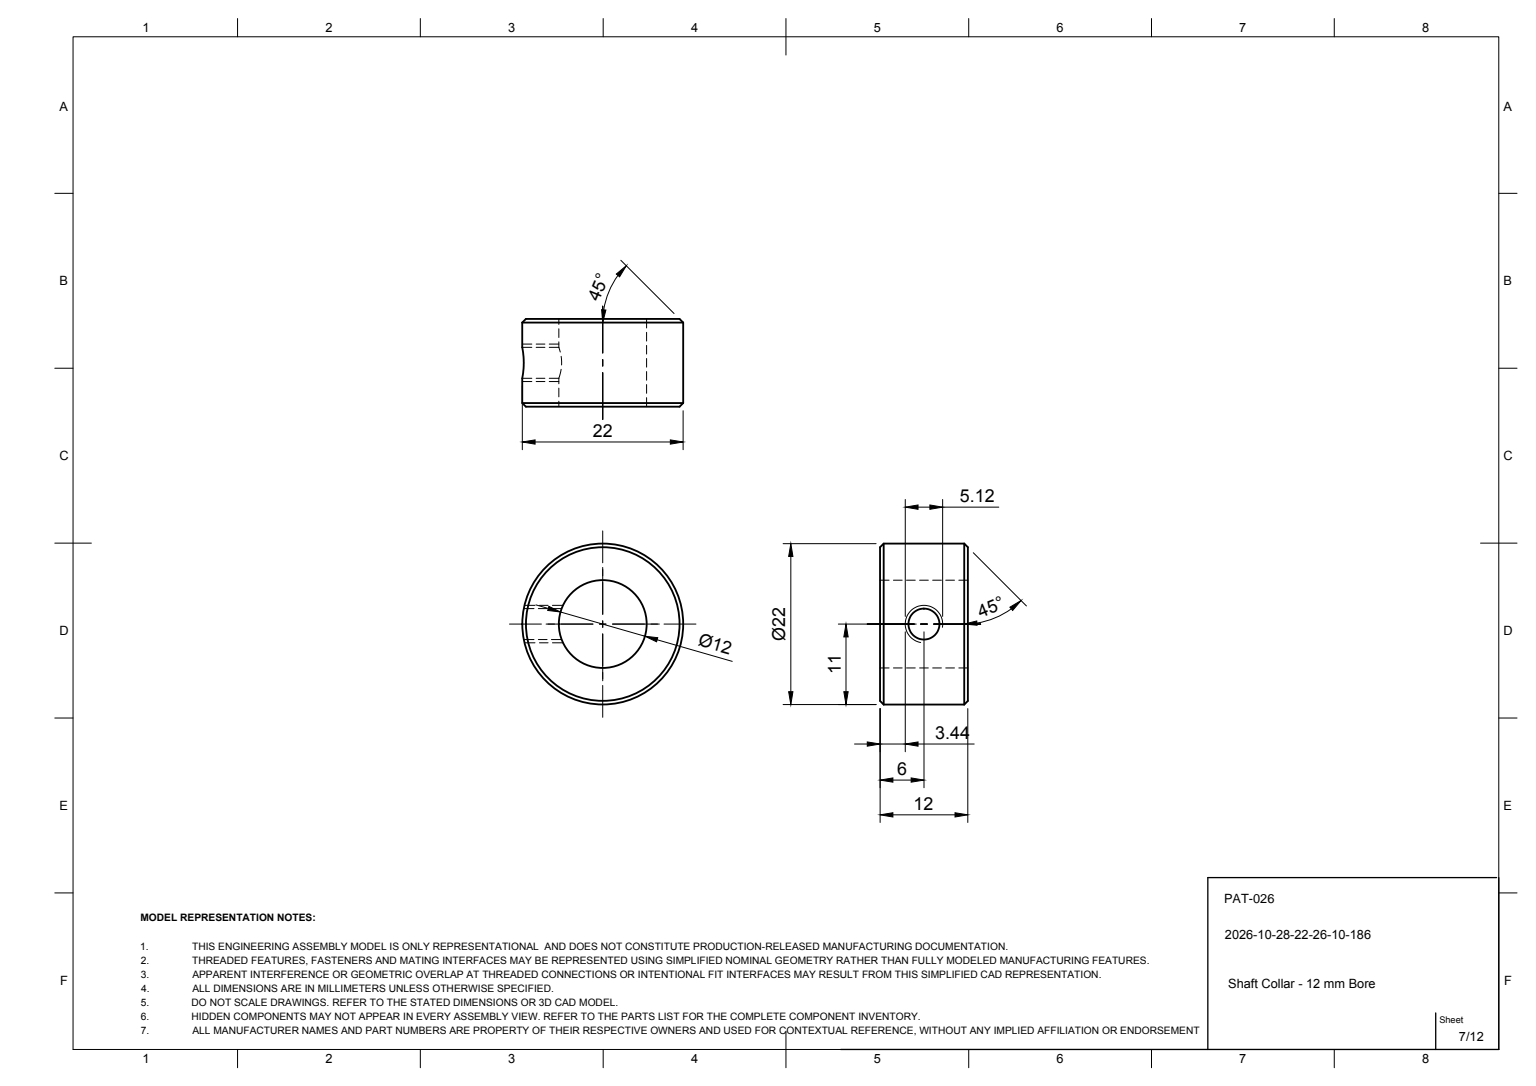
ISO-10303-21;
HEADER;
/* Generated by software containing ST-Developer
 * from STEP Tools, Inc. (www.steptools.com) 
 */

FILE_DESCRIPTION(
/* description */ ('PAT-026'),
/* implementation_level */ '2;1');

FILE_NAME(
/* name */ 'Shaft Collar - 12 mm Bore.step',
/* time_stamp */ '2026-10-28T22:25:58-07:00',
/* author */ (''),
/* organization */ (''),
/* preprocessor_version */ 'ST-DEVELOPER v20.2',
/* originating_system */ 'Autodesk Translation Framework v15.17.0.0',
/* authorisation */ '');

FILE_SCHEMA (('AUTOMOTIVE_DESIGN { 1 0 10303 214 3 1 1 }'));
ENDSEC;

DATA;
#10=MECHANICAL_DESIGN_GEOMETRIC_PRESENTATION_REPRESENTATION('',(#147),#12343);
#95=B_SPLINE_CURVE_WITH_KNOTS('',3,(#10378,#10379,#10380,#10381,#10382,
#10383,#10384,#10385,#10386,#10387,#10388,#10389,#10390,#10391,#10392,#10393,
#10394,#10395,#10396,#10397,#10398,#10399,#10400,#10401,#10402,#10403,#10404,
#10405,#10406,#10407,#10408,#10409,#10410,#10411),.UNSPECIFIED.,.T.,.F.,
(4,2,2,2,2,2,2,2,2,2,2,2,2,2,2,2,4),(0.,0.0805240527913139,0.161048105582628,
0.241524630728584,0.322001155874541,0.402477681020498,0.482954206166455,
0.563478258957768,0.644002311749082,0.724526364540396,0.80505041733171,
0.885526942477667,0.966003467623624,1.04647999276958,1.12695651791554,1.20748057070685,
1.28800462349816),.UNSPECIFIED.);
#96=B_SPLINE_CURVE_WITH_KNOTS('',3,(#10414,#10415,#10416,#10417,#10418,
#10419,#10420,#10421,#10422,#10423,#10424,#10425,#10426,#10427,#10428,#10429,
#10430,#10431,#10432,#10433,#10434,#10435,#10436,#10437,#10438,#10439,#10440,
#10441,#10442,#10443,#10444,#10445,#10446,#10447),.UNSPECIFIED.,.T.,.F.,
(4,2,2,2,2,2,2,2,2,2,2,2,2,2,2,2,4),(0.,0.0799614062161292,0.159922812432258,
0.239880387792505,0.319837963152752,0.399795538512999,0.479753113873245,
0.559714520089374,0.639675926305503,0.719637332521632,0.799598738737761,
0.879556314098008,0.959513889458255,1.0394714648185,1.11942904017875,1.19939044639488,
1.27935185261101),.UNSPECIFIED.);
#111=CONICAL_SURFACE('',#7607,1.075,0.785398163397448);
#112=CONICAL_SURFACE('',#7611,1.075,0.785398163397449);
#125=SHAPE_REPRESENTATION_RELATIONSHIP('SRR','None',#12402,#136);
#136=ADVANCED_BREP_SHAPE_REPRESENTATION('',(#156),#12337);
#147=STYLED_ITEM('',(#12533),#156);
#156=MANIFOLD_SOLID_BREP('Body1',#7355);
#181=FACE_BOUND('',#1050,.T.);
#182=FACE_BOUND('',#1053,.T.);
#183=FACE_BOUND('',#1056,.T.);
#184=FACE_BOUND('',#1058,.T.);
#242=PLANE('',#7604);
#243=PLANE('',#7613);
#625=FACE_OUTER_BOUND('',#1048,.T.);
#626=FACE_OUTER_BOUND('',#1049,.T.);
#627=FACE_OUTER_BOUND('',#1051,.T.);
#628=FACE_OUTER_BOUND('',#1052,.T.);
#629=FACE_OUTER_BOUND('',#1054,.T.);
#630=FACE_OUTER_BOUND('',#1055,.T.);
#631=FACE_OUTER_BOUND('',#1057,.T.);
#1048=EDGE_LOOP('',(#5209,#5210,#5211,#5212));
#1049=EDGE_LOOP('',(#5213));
#1050=EDGE_LOOP('',(#5214));
#1051=EDGE_LOOP('',(#5215,#5216,#5217,#5218));
#1052=EDGE_LOOP('',(#5219,#5220,#5221,#5222));
#1053=EDGE_LOOP('',(#5223));
#1054=EDGE_LOOP('',(#5224,#5225,#5226,#5227));
#1055=EDGE_LOOP('',(#5228));
#1056=EDGE_LOOP('',(#5229));
#1057=EDGE_LOOP('',(#5230,#5231,#5232,#5233));
#1058=EDGE_LOOP('',(#5234));
#1506=LINE('',#10413,#2378);
#1507=LINE('',#10456,#2379);
#1508=LINE('',#10460,#2380);
#1509=LINE('',#10464,#2381);
#1510=LINE('',#10469,#2382);
#2378=VECTOR('',#8402,0.21);
#2379=VECTOR('',#8413,1.075);
#2380=VECTOR('',#8418,1.1);
#2381=VECTOR('',#8423,1.075);
#2382=VECTOR('',#8430,0.6);
#3177=CIRCLE('',#7605,1.05);
#3178=CIRCLE('',#7606,0.6);
#3179=CIRCLE('',#7608,1.1);
#3180=CIRCLE('',#7610,1.1);
#3181=CIRCLE('',#7612,1.05);
#3182=CIRCLE('',#7614,0.6);
#3362=VERTEX_POINT('',#10377);
#3363=VERTEX_POINT('',#10412);
#3364=VERTEX_POINT('',#10449);
#3365=VERTEX_POINT('',#10451);
#3366=VERTEX_POINT('',#10454);
#3367=VERTEX_POINT('',#10458);
#3368=VERTEX_POINT('',#10462);
#3369=VERTEX_POINT('',#10466);
#4048=EDGE_CURVE('',#3362,#3362,#95,.T.);
#4049=EDGE_CURVE('',#3362,#3363,#1506,.T.);
#4050=EDGE_CURVE('',#3363,#3363,#96,.T.);
#4051=EDGE_CURVE('',#3364,#3364,#3177,.T.);
#4052=EDGE_CURVE('',#3365,#3365,#3178,.T.);
#4053=EDGE_CURVE('',#3366,#3366,#3179,.T.);
#4054=EDGE_CURVE('',#3366,#3364,#1507,.T.);
#4055=EDGE_CURVE('',#3367,#3367,#3180,.T.);
#4056=EDGE_CURVE('',#3367,#3366,#1508,.T.);
#4057=EDGE_CURVE('',#3368,#3368,#3181,.T.);
#4058=EDGE_CURVE('',#3368,#3367,#1509,.T.);
#4059=EDGE_CURVE('',#3369,#3369,#3182,.T.);
#4060=EDGE_CURVE('',#3369,#3365,#1510,.T.);
#5209=ORIENTED_EDGE('',*,*,#4048,.F.);
#5210=ORIENTED_EDGE('',*,*,#4049,.T.);
#5211=ORIENTED_EDGE('',*,*,#4050,.F.);
#5212=ORIENTED_EDGE('',*,*,#4049,.F.);
#5213=ORIENTED_EDGE('',*,*,#4051,.F.);
#5214=ORIENTED_EDGE('',*,*,#4052,.T.);
#5215=ORIENTED_EDGE('',*,*,#4053,.F.);
#5216=ORIENTED_EDGE('',*,*,#4054,.T.);
#5217=ORIENTED_EDGE('',*,*,#4051,.T.);
#5218=ORIENTED_EDGE('',*,*,#4054,.F.);
#5219=ORIENTED_EDGE('',*,*,#4055,.F.);
#5220=ORIENTED_EDGE('',*,*,#4056,.T.);
#5221=ORIENTED_EDGE('',*,*,#4053,.T.);
#5222=ORIENTED_EDGE('',*,*,#4056,.F.);
#5223=ORIENTED_EDGE('',*,*,#4050,.T.);
#5224=ORIENTED_EDGE('',*,*,#4057,.F.);
#5225=ORIENTED_EDGE('',*,*,#4058,.T.);
#5226=ORIENTED_EDGE('',*,*,#4055,.T.);
#5227=ORIENTED_EDGE('',*,*,#4058,.F.);
#5228=ORIENTED_EDGE('',*,*,#4057,.T.);
#5229=ORIENTED_EDGE('',*,*,#4059,.F.);
#5230=ORIENTED_EDGE('',*,*,#4059,.T.);
#5231=ORIENTED_EDGE('',*,*,#4060,.T.);
#5232=ORIENTED_EDGE('',*,*,#4052,.F.);
#5233=ORIENTED_EDGE('',*,*,#4060,.F.);
#5234=ORIENTED_EDGE('',*,*,#4048,.T.);
#6928=CYLINDRICAL_SURFACE('',#7603,0.2117);
#6929=CYLINDRICAL_SURFACE('',#7609,1.1);
#6930=CYLINDRICAL_SURFACE('',#7615,0.6);
#7016=ADVANCED_FACE('',(#625),#6928,.F.);
#7017=ADVANCED_FACE('',(#626,#181),#242,.T.);
#7018=ADVANCED_FACE('',(#627),#111,.T.);
#7019=ADVANCED_FACE('',(#628,#182),#6929,.T.);
#7020=ADVANCED_FACE('',(#629),#112,.T.);
#7021=ADVANCED_FACE('',(#630,#183),#243,.T.);
#7022=ADVANCED_FACE('',(#631,#184),#6930,.F.);
#7355=CLOSED_SHELL('',(#7016,#7017,#7018,#7019,#7020,#7021,#7022));
#7602=AXIS2_PLACEMENT_3D('',#10375,#8398,#8399);
#7603=AXIS2_PLACEMENT_3D('',#10376,#8400,#8401);
#7604=AXIS2_PLACEMENT_3D('',#10448,#8403,#8404);
#7605=AXIS2_PLACEMENT_3D('',#10450,#8405,#8406);
#7606=AXIS2_PLACEMENT_3D('',#10452,#8407,#8408);
#7607=AXIS2_PLACEMENT_3D('',#10453,#8409,#8410);
#7608=AXIS2_PLACEMENT_3D('',#10455,#8411,#8412);
#7609=AXIS2_PLACEMENT_3D('',#10457,#8414,#8415);
#7610=AXIS2_PLACEMENT_3D('',#10459,#8416,#8417);
#7611=AXIS2_PLACEMENT_3D('',#10461,#8419,#8420);
#7612=AXIS2_PLACEMENT_3D('',#10463,#8421,#8422);
#7613=AXIS2_PLACEMENT_3D('',#10465,#8424,#8425);
#7614=AXIS2_PLACEMENT_3D('',#10467,#8426,#8427);
#7615=AXIS2_PLACEMENT_3D('',#10468,#8428,#8429);
#8398=DIRECTION('axis',(0.,0.,1.));
#8399=DIRECTION('refdir',(1.,0.,0.));
#8400=DIRECTION('center_axis',(1.,0.,0.));
#8401=DIRECTION('ref_axis',(0.,0.,-1.));
#8402=DIRECTION('',(1.,0.,0.));
#8403=DIRECTION('center_axis',(0.,1.,0.));
#8404=DIRECTION('ref_axis',(0.,0.,1.));
#8405=DIRECTION('center_axis',(0.,-1.,0.));
#8406=DIRECTION('ref_axis',(1.,0.,0.));
#8407=DIRECTION('center_axis',(0.,-1.,0.));
#8408=DIRECTION('ref_axis',(1.,0.,0.));
#8409=DIRECTION('center_axis',(0.,-1.,0.));
#8410=DIRECTION('ref_axis',(1.,0.,0.));
#8411=DIRECTION('center_axis',(0.,-1.,0.));
#8412=DIRECTION('ref_axis',(1.,0.,0.));
#8413=DIRECTION('',(0.707106781186548,0.707106781186547,8.65956056235493E-17));
#8414=DIRECTION('center_axis',(0.,-1.,0.));
#8415=DIRECTION('ref_axis',(1.,0.,0.));
#8416=DIRECTION('center_axis',(0.,-1.,0.));
#8417=DIRECTION('ref_axis',(1.,0.,0.));
#8418=DIRECTION('',(0.,1.,0.));
#8419=DIRECTION('center_axis',(0.,1.,0.));
#8420=DIRECTION('ref_axis',(1.,0.,0.));
#8421=DIRECTION('center_axis',(0.,-1.,0.));
#8422=DIRECTION('ref_axis',(1.,0.,0.));
#8423=DIRECTION('',(-0.707106781186548,0.707106781186547,-8.65956056235494E-17));
#8424=DIRECTION('center_axis',(0.,-1.,0.));
#8425=DIRECTION('ref_axis',(0.,0.,-1.));
#8426=DIRECTION('center_axis',(0.,-1.,0.));
#8427=DIRECTION('ref_axis',(1.,0.,0.));
#8428=DIRECTION('center_axis',(0.,-1.,0.));
#8429=DIRECTION('ref_axis',(1.,0.,0.));
#8430=DIRECTION('',(0.,1.,0.));
#10375=CARTESIAN_POINT('',(0.,0.,0.));
#10376=CARTESIAN_POINT('Origin',(0.5,0.6,0.));
#10377=CARTESIAN_POINT('',(0.561411711669787,0.6,0.2117));
#10378=CARTESIAN_POINT('Ctrl Pts',(0.561411711669787,0.6,0.2117));
#10379=CARTESIAN_POINT('Ctrl Pts',(0.561411711669787,0.573158649069562,
0.2117));
#10380=CARTESIAN_POINT('Ctrl Pts',(0.563539297838208,0.544705001203387,
0.206288194517509));
#10381=CARTESIAN_POINT('Ctrl Pts',(0.571006257413022,0.492626080621549,
0.184616375754799));
#10382=CARTESIAN_POINT('Ctrl Pts',(0.576215579648966,0.468977868958045,
0.168366880112429));
#10383=CARTESIAN_POINT('Ctrl Pts',(0.585834170098139,0.431644140867814,
0.131033152022198));
#10384=CARTESIAN_POINT('Ctrl Pts',(0.590898115435695,0.41538619377614,0.107380608633747));
#10385=CARTESIAN_POINT('Ctrl Pts',(0.598025669508798,0.393708029332882,
0.0552854099234836));
#10386=CARTESIAN_POINT('Ctrl Pts',(0.6,0.3883,0.0268255083819855));
#10387=CARTESIAN_POINT('Ctrl Pts',(0.6,0.3883,-0.0268255083819856));
#10388=CARTESIAN_POINT('Ctrl Pts',(0.598025669508798,0.393708029332882,
-0.0552854099234837));
#10389=CARTESIAN_POINT('Ctrl Pts',(0.590898115435695,0.41538619377614,-0.107380608633747));
#10390=CARTESIAN_POINT('Ctrl Pts',(0.585834170098139,0.431644140867814,
-0.131033152022198));
#10391=CARTESIAN_POINT('Ctrl Pts',(0.576215579648966,0.468977868958045,
-0.168366880112429));
#10392=CARTESIAN_POINT('Ctrl Pts',(0.571006257413022,0.49262608062155,-0.184616375754799));
#10393=CARTESIAN_POINT('Ctrl Pts',(0.563539297838207,0.544705001203387,
-0.206288194517509));
#10394=CARTESIAN_POINT('Ctrl Pts',(0.561411711669787,0.573158649069562,
-0.2117));
#10395=CARTESIAN_POINT('Ctrl Pts',(0.561411711669787,0.626841350930438,
-0.2117));
#10396=CARTESIAN_POINT('Ctrl Pts',(0.563539297838207,0.655294998796613,
-0.206288194517509));
#10397=CARTESIAN_POINT('Ctrl Pts',(0.571006257413022,0.70737391937845,-0.184616375754799));
#10398=CARTESIAN_POINT('Ctrl Pts',(0.576215579648966,0.731022131041955,
-0.168366880112429));
#10399=CARTESIAN_POINT('Ctrl Pts',(0.585834170098139,0.768355859132186,
-0.131033152022198));
#10400=CARTESIAN_POINT('Ctrl Pts',(0.590898115435695,0.78461380622386,-0.107380608633747));
#10401=CARTESIAN_POINT('Ctrl Pts',(0.598025669508798,0.806291970667118,
-0.0552854099234837));
#10402=CARTESIAN_POINT('Ctrl Pts',(0.6,0.8117,-0.0268255083819856));
#10403=CARTESIAN_POINT('Ctrl Pts',(0.6,0.8117,0.0268255083819855));
#10404=CARTESIAN_POINT('Ctrl Pts',(0.598025669508798,0.806291970667118,
0.0552854099234837));
#10405=CARTESIAN_POINT('Ctrl Pts',(0.590898115435695,0.78461380622386,0.107380608633747));
#10406=CARTESIAN_POINT('Ctrl Pts',(0.585834170098139,0.768355859132186,
0.131033152022198));
#10407=CARTESIAN_POINT('Ctrl Pts',(0.576215579648966,0.731022131041955,
0.168366880112429));
#10408=CARTESIAN_POINT('Ctrl Pts',(0.571006257413022,0.70737391937845,0.184616375754799));
#10409=CARTESIAN_POINT('Ctrl Pts',(0.563539297838207,0.655294998796613,
0.206288194517509));
#10410=CARTESIAN_POINT('Ctrl Pts',(0.561411711669787,0.626841350930438,
0.2117));
#10411=CARTESIAN_POINT('Ctrl Pts',(0.561411711669787,0.6,0.2117));
#10412=CARTESIAN_POINT('',(1.07943647798284,0.6,0.2117));
#10413=CARTESIAN_POINT('',(0.5,0.6,0.2117));
#10414=CARTESIAN_POINT('Ctrl Pts',(1.07943647798284,0.6,0.2117));
#10415=CARTESIAN_POINT('Ctrl Pts',(1.07943647798284,0.626653802072043,0.2117));
#10416=CARTESIAN_POINT('Ctrl Pts',(1.08052600621577,0.655037401084091,0.206359582618511));
#10417=CARTESIAN_POINT('Ctrl Pts',(1.08443252298676,0.707175401021015,0.18473448130117));
#10418=CARTESIAN_POINT('Ctrl Pts',(1.08718996287164,0.730935702749545,0.168453308404839));
#10419=CARTESIAN_POINT('Ctrl Pts',(1.09234340045893,0.768452409692904,0.13093660146148));
#10420=CARTESIAN_POINT('Ctrl Pts',(1.09507838311905,0.784734286816328,0.107175917083711));
#10421=CARTESIAN_POINT('Ctrl Pts',(1.09893326276149,0.806359899102434,0.0550365908820453));
#10422=CARTESIAN_POINT('Ctrl Pts',(1.1,0.8117,0.0266525251200821));
#10423=CARTESIAN_POINT('Ctrl Pts',(1.1,0.8117,-0.0266525251200823));
#10424=CARTESIAN_POINT('Ctrl Pts',(1.09893326276149,0.806359899102434,-0.0550365908820454));
#10425=CARTESIAN_POINT('Ctrl Pts',(1.09507838311905,0.784734286816328,-0.107175917083711));
#10426=CARTESIAN_POINT('Ctrl Pts',(1.09234340045893,0.768452409692904,-0.130936601461481));
#10427=CARTESIAN_POINT('Ctrl Pts',(1.08718996287164,0.730935702749545,-0.16845330840484));
#10428=CARTESIAN_POINT('Ctrl Pts',(1.08443252298676,0.707175401021015,-0.18473448130117));
#10429=CARTESIAN_POINT('Ctrl Pts',(1.08052600621577,0.655037401084091,-0.206359582618511));
#10430=CARTESIAN_POINT('Ctrl Pts',(1.07943647798284,0.626653802072043,-0.2117));
#10431=CARTESIAN_POINT('Ctrl Pts',(1.07943647798284,0.573346197927957,-0.2117));
#10432=CARTESIAN_POINT('Ctrl Pts',(1.08052600621577,0.544962598915909,-0.206359582618511));
#10433=CARTESIAN_POINT('Ctrl Pts',(1.08443252298676,0.492824598978985,-0.18473448130117));
#10434=CARTESIAN_POINT('Ctrl Pts',(1.08718996287164,0.469064297250455,-0.168453308404839));
#10435=CARTESIAN_POINT('Ctrl Pts',(1.09234340045893,0.431547590307096,-0.13093660146148));
#10436=CARTESIAN_POINT('Ctrl Pts',(1.09507838311905,0.415265713183672,-0.107175917083711));
#10437=CARTESIAN_POINT('Ctrl Pts',(1.09893326276149,0.393640100897566,-0.0550365908820454));
#10438=CARTESIAN_POINT('Ctrl Pts',(1.1,0.3883,-0.0266525251200822));
#10439=CARTESIAN_POINT('Ctrl Pts',(1.1,0.3883,0.0266525251200823));
#10440=CARTESIAN_POINT('Ctrl Pts',(1.09893326276149,0.393640100897566,0.0550365908820454));
#10441=CARTESIAN_POINT('Ctrl Pts',(1.09507838311905,0.415265713183672,0.107175917083711));
#10442=CARTESIAN_POINT('Ctrl Pts',(1.09234340045893,0.431547590307096,0.13093660146148));
#10443=CARTESIAN_POINT('Ctrl Pts',(1.08718996287164,0.469064297250455,0.16845330840484));
#10444=CARTESIAN_POINT('Ctrl Pts',(1.08443252298676,0.492824598978985,0.18473448130117));
#10445=CARTESIAN_POINT('Ctrl Pts',(1.08052600621577,0.544962598915909,0.206359582618511));
#10446=CARTESIAN_POINT('Ctrl Pts',(1.07943647798284,0.573346197927957,0.2117));
#10447=CARTESIAN_POINT('Ctrl Pts',(1.07943647798284,0.6,0.2117));
#10448=CARTESIAN_POINT('Origin',(1.05,1.2,0.));
#10449=CARTESIAN_POINT('',(-1.05,1.2,-1.28587913910472E-16));
#10450=CARTESIAN_POINT('Origin',(0.,1.2,0.));
#10451=CARTESIAN_POINT('',(-0.6,1.2,-7.34788079488412E-17));
#10452=CARTESIAN_POINT('Origin',(0.,1.2,0.));
#10453=CARTESIAN_POINT('Origin',(0.,1.175,0.));
#10454=CARTESIAN_POINT('',(-1.1,1.15,-1.34711147906209E-16));
#10455=CARTESIAN_POINT('Origin',(0.,1.15,0.));
#10456=CARTESIAN_POINT('',(-1.075,1.175,-1.3164953090834E-16));
#10457=CARTESIAN_POINT('Origin',(0.,0.6,0.));
#10458=CARTESIAN_POINT('',(-1.1,0.05,-1.34711147906209E-16));
#10459=CARTESIAN_POINT('Origin',(0.,0.05,0.));
#10460=CARTESIAN_POINT('',(-1.1,0.6,-1.34711147906209E-16));
#10461=CARTESIAN_POINT('Origin',(0.,0.025,0.));
#10462=CARTESIAN_POINT('',(-1.05,-4.5102810375397E-17,-1.28587913910472E-16));
#10463=CARTESIAN_POINT('Origin',(0.,0.,0.));
#10464=CARTESIAN_POINT('',(-1.075,0.025,-1.3164953090834E-16));
#10465=CARTESIAN_POINT('Origin',(0.6,0.,0.));
#10466=CARTESIAN_POINT('',(-0.6,0.,-7.34788079488412E-17));
#10467=CARTESIAN_POINT('Origin',(0.,0.,0.));
#10468=CARTESIAN_POINT('Origin',(0.,0.6,0.));
#10469=CARTESIAN_POINT('',(-0.6,0.6,-7.34788079488412E-17));
#12323=UNCERTAINTY_MEASURE_WITH_UNIT(LENGTH_MEASURE(0.001),#12344,
'DISTANCE_ACCURACY_VALUE',
'Maximum model space distance between geometric entities at asserted c
onnectivities');
#12329=UNCERTAINTY_MEASURE_WITH_UNIT(LENGTH_MEASURE(0.001),#12344,
'DISTANCE_ACCURACY_VALUE',
'Maximum model space distance between geometric entities at asserted c
onnectivities');
#12337=(
GEOMETRIC_REPRESENTATION_CONTEXT(3)
GLOBAL_UNCERTAINTY_ASSIGNED_CONTEXT((#12323))
GLOBAL_UNIT_ASSIGNED_CONTEXT((#12344,#12346,#12347))
REPRESENTATION_CONTEXT('','3D')
);
#12343=(
GEOMETRIC_REPRESENTATION_CONTEXT(3)
GLOBAL_UNCERTAINTY_ASSIGNED_CONTEXT((#12329))
GLOBAL_UNIT_ASSIGNED_CONTEXT((#12344,#12346,#12347))
REPRESENTATION_CONTEXT('','3D')
);
#12344=(
LENGTH_UNIT()
NAMED_UNIT(*)
SI_UNIT(.CENTI.,.METRE.)
);
#12346=(
NAMED_UNIT(*)
PLANE_ANGLE_UNIT()
SI_UNIT($,.RADIAN.)
);
#12347=(
NAMED_UNIT(*)
SI_UNIT($,.STERADIAN.)
SOLID_ANGLE_UNIT()
);
#12355=SHAPE_DEFINITION_REPRESENTATION(#12368,#12402);
#12368=PRODUCT_DEFINITION_SHAPE('',$,#12416);
#12402=SHAPE_REPRESENTATION('',(#7602),#12337);
#12408=PRODUCT_DEFINITION_CONTEXT('part definition',#12449,'design');
#12416=PRODUCT_DEFINITION('Shaft Collar - 12 mm Bore',
'Shaft Collar - 12 mm Bore',#12429,#12408);
#12429=PRODUCT_DEFINITION_FORMATION('',$,#12458);
#12449=APPLICATION_CONTEXT(
'Core Data for Automotive Mechanical Design Process');
#12450=PRODUCT_CONTEXT('part definition',#12449,'mechanical');
#12458=PRODUCT('Shaft Collar - 12 mm Bore','Shaft Collar - 12 mm Bore',
'Shaft Collar - 12 mm Bore',(#12450));
#12527=COLOUR_RGB('Grey',0.48,0.52,0.57);
#12528=FILL_AREA_STYLE_COLOUR('',#12527);
#12529=FILL_AREA_STYLE('',(#12528));
#12530=SURFACE_STYLE_FILL_AREA(#12529);
#12531=SURFACE_SIDE_STYLE('',(#12530));
#12532=SURFACE_STYLE_USAGE(.BOTH.,#12531);
#12533=PRESENTATION_STYLE_ASSIGNMENT((#12532));
ENDSEC;
END-ISO-10303-21;
